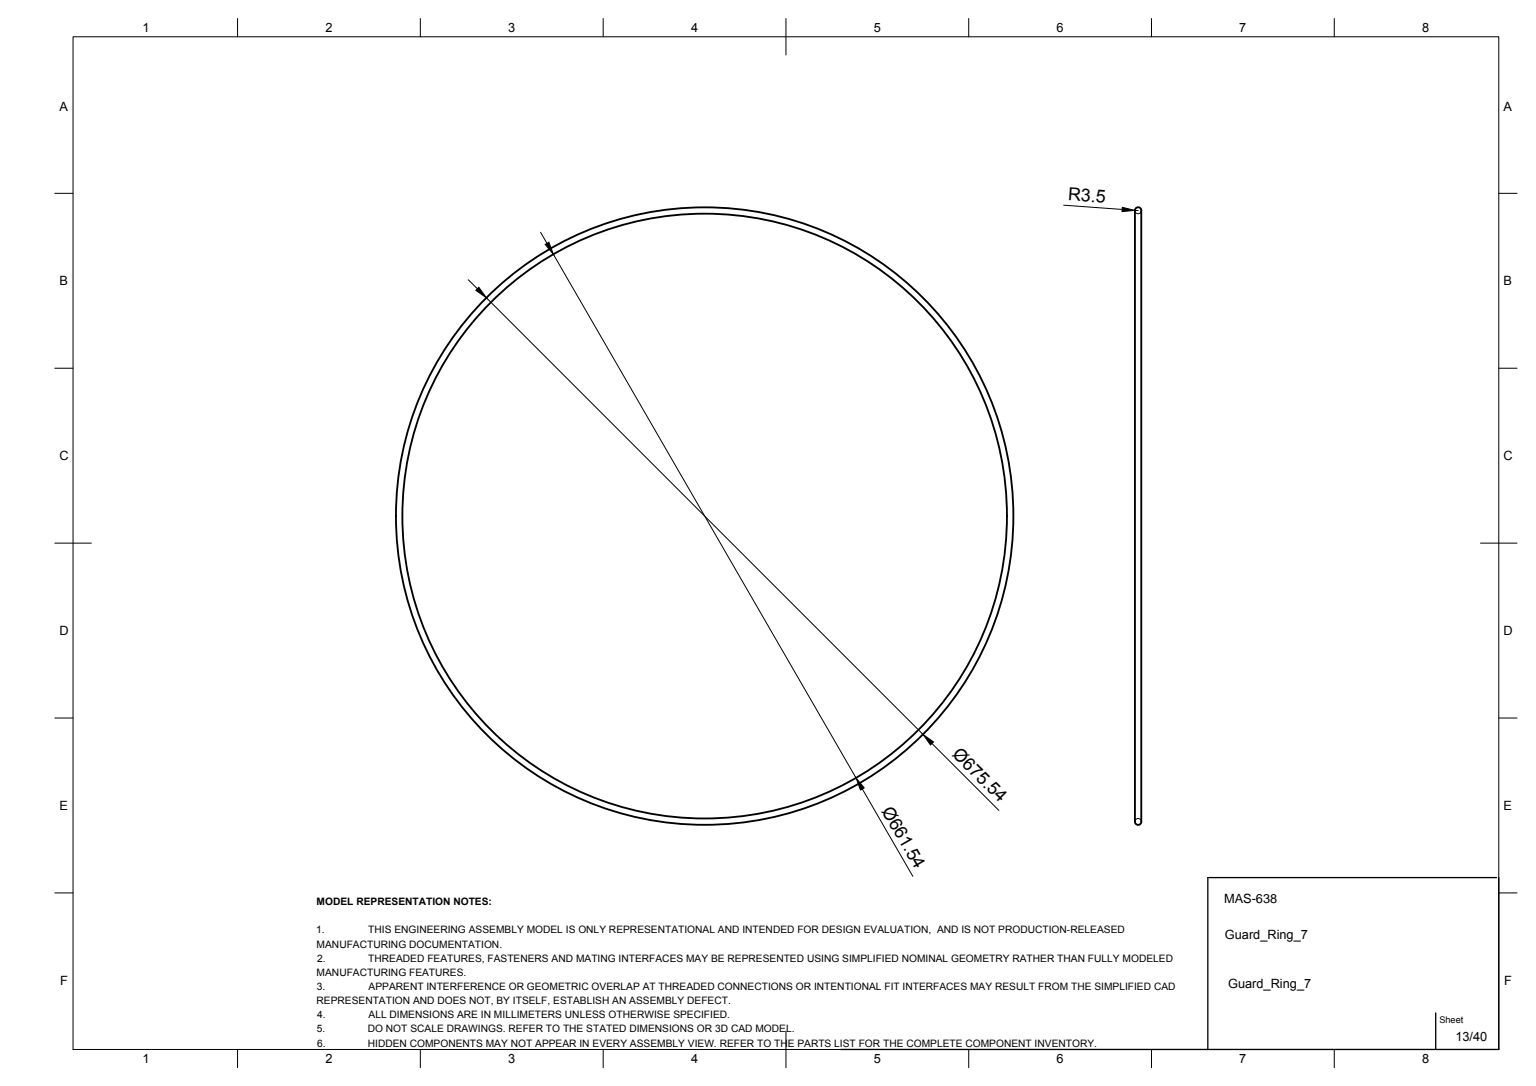
ISO-10303-21;
HEADER;
FILE_DESCRIPTION((''),'2;1');
FILE_NAME('Guard_Ring_7.step','2026-10-09T12:00:21-07:00',(''),(''),'','','');
FILE_SCHEMA (('AUTOMOTIVE_DESIGN { 1 0 10303 214 3 1 1 }'));
ENDSEC;
DATA;
#10=MECHANICAL_DESIGN_GEOMETRIC_PRESENTATION_REPRESENTATION('',(#404),#10334);
#340=SHAPE_REPRESENTATION_RELATIONSHIP('SRR','None',#10456,#372) ;
#372=ADVANCED_BREP_SHAPE_REPRESENTATION('',(#444),#10308) ;
#404=STYLED_ITEM('',(#10631),#444) ;
#444=MANIFOLD_SOLID_BREP('Body1',#3566) ;
#865=FACE_OUTER_BOUND('',#1065,.T.) ;
#1065=EDGE_LOOP('',(#2373,#2374,#2375,#2376)) ;
#1288=CIRCLE('',#3999,0.349999999999999) ;
#1289=CIRCLE('',#4000,33.0768144613668) ;
#1519=VERTEX_POINT('',#5683) ;
#1843=EDGE_CURVE('',#1519,#1519,#1288,.T.) ;
#1844=EDGE_CURVE('',#1519,#1519,#1289,.T.) ;
#2373=ORIENTED_EDGE('',*,*,#1843,.F.) ;
#2374=ORIENTED_EDGE('',*,*,#1844,.T.) ;
#2375=ORIENTED_EDGE('',*,*,#1843,.T.) ;
#2376=ORIENTED_EDGE('',*,*,#1844,.F.) ;
#3311=TOROIDAL_SURFACE('',#3998,33.4268144613668,0.349999999999999) ;
#3373=ADVANCED_FACE('',(#865),#3311,.T.) ;
#3566=CLOSED_SHELL('',(#3373)) ;
#3997=AXIS2_PLACEMENT_3D('',#5681,#4555,#4556) ;
#3998=AXIS2_PLACEMENT_3D('',#5682,#4557,#4558) ;
#3999=AXIS2_PLACEMENT_3D('',#5684,#4559,#4560) ;
#4000=AXIS2_PLACEMENT_3D('',#5685,#4561,#4562) ;
#4555=DIRECTION('axis',(0.,0.,1.)) ;
#4556=DIRECTION('refdir',(1.,0.,0.)) ;
#4557=DIRECTION('center_axis',(-6.42891162084177E-17,-1.,-1.01883556321148E-16)) ;
#4558=DIRECTION('ref_axis',(1.,0.,0.)) ;
#4559=DIRECTION('center_axis',(0.,1.01883556321148E-16,-1.)) ;
#4560=DIRECTION('ref_axis',(-1.,0.,0.)) ;
#4561=DIRECTION('center_axis',(6.42891162084177E-17,1.,1.01883556321148E-16)) ;
#4562=DIRECTION('ref_axis',(1.,-6.42891162084177E-17,-6.55000379205715E-33)) ;
#5681=CARTESIAN_POINT('',(0.,0.,0.)) ;
#5682=CARTESIAN_POINT('Origin',(23.47768801576,67.3831179463143,68.2224337400009)) ;
#5683=CARTESIAN_POINT('',(-9.5991264456068,67.3831179463143,68.2224337400009)) ;
#5684=CARTESIAN_POINT('Origin',(-9.9491264456068,67.3831179463143,68.2224337400009)) ;
#5685=CARTESIAN_POINT('Origin',(23.47768801576,67.3831179463143,68.2224337400009)) ;
#10271=UNCERTAINTY_MEASURE_WITH_UNIT(LENGTH_MEASURE(0.001),#10335,
'DISTANCE_ACCURACY_VALUE',
'Maximum model space distance between geometric entities at asserted c
onnectivities') ;
#10297=UNCERTAINTY_MEASURE_WITH_UNIT(LENGTH_MEASURE(0.001),#10335,
'DISTANCE_ACCURACY_VALUE',
'Maximum model space distance between geometric entities at asserted c
onnectivities') ;
#10308=(
GEOMETRIC_REPRESENTATION_CONTEXT(3)
GLOBAL_UNCERTAINTY_ASSIGNED_CONTEXT((#10271))
GLOBAL_UNIT_ASSIGNED_CONTEXT((#10335,#10337,#10338))
REPRESENTATION_CONTEXT('','3D')
) ;
#10334=(
GEOMETRIC_REPRESENTATION_CONTEXT(3)
GLOBAL_UNCERTAINTY_ASSIGNED_CONTEXT((#10297))
GLOBAL_UNIT_ASSIGNED_CONTEXT((#10335,#10337,#10338))
REPRESENTATION_CONTEXT('','3D')
) ;
#10335=(
LENGTH_UNIT()
NAMED_UNIT(*)
SI_UNIT(.CENTI.,.METRE.)
) ;
#10337=(
NAMED_UNIT(*)
PLANE_ANGLE_UNIT()
SI_UNIT($,.RADIAN.)
) ;
#10338=(
NAMED_UNIT(*)
SI_UNIT($,.STERADIAN.)
SOLID_ANGLE_UNIT()
) ;
#10349=SHAPE_DEFINITION_REPRESENTATION(#10385,#10456) ;
#10385=PRODUCT_DEFINITION_SHAPE('',$,#10493) ;
#10456=SHAPE_REPRESENTATION('',(#3997),#10308) ;
#10482=PRODUCT_DEFINITION_CONTEXT('part definition',#10592,'design') ;
#10493=PRODUCT_DEFINITION('Guard_Ring_7','Guard_Ring_7',#10529,#10482) ;
#10529=PRODUCT_DEFINITION_FORMATION('',$,#10604) ;
#10592=APPLICATION_CONTEXT(
'Core Data for Automotive Mechanical Design Process') ;
#10593=PRODUCT_CONTEXT('part definition',#10592,'mechanical') ;
#10604=PRODUCT('Guard_Ring_7','Guard_Ring_7',$,(#10593)) ;
#10631=PRESENTATION_STYLE_ASSIGNMENT((#10635)) ;
#10635=SURFACE_STYLE_USAGE(.BOTH.,#10639) ;
#10639=SURFACE_SIDE_STYLE('',(#10643)) ;
#10643=SURFACE_STYLE_FILL_AREA(#10647) ;
#10647=FILL_AREA_STYLE('Opaque(25,25,25)',(#10651)) ;
#10651=FILL_AREA_STYLE_COLOUR('Opaque(25,25,25)',#10655) ;
#10655=COLOUR_RGB('Opaque(25,25,25)', 0.09019608, 0.27058824, 0.51372549) ;
ENDSEC;
END-ISO-10303-21;
